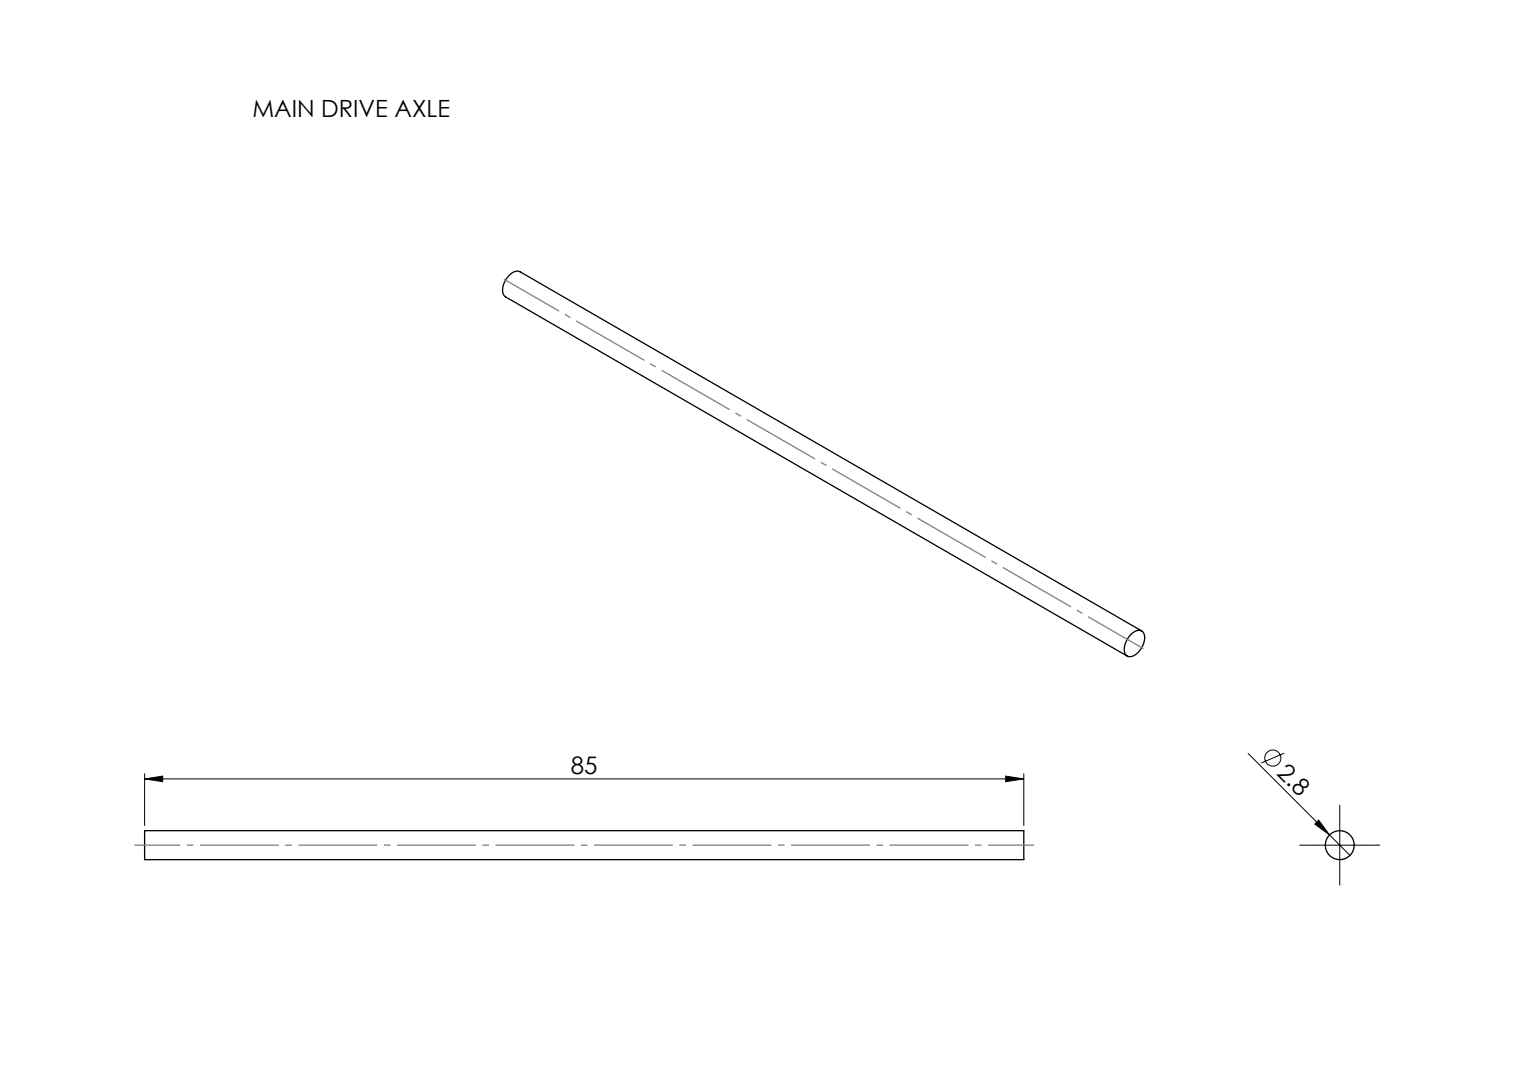
ISO-10303-21;
HEADER;
FILE_DESCRIPTION (('STEP AP214'),
    '1' );
FILE_NAME ('main drive axle.step',
    '2026-10-09T15:17:24',
    ( '' ),
    ( '' ),
    'SwSTEP 2.0',
    'SolidWorks 2026',
    '' );
FILE_SCHEMA (( 'AUTOMOTIVE_DESIGN' ));
ENDSEC;

DATA;
#499=ORIENTED_EDGE ( 'NONE', *, *, #57601, .F. ) ;
#808=LINE ( 'NONE', #11431, #63431 ) ;
#1848=CARTESIAN_POINT ( 'NONE',  ( 42.50000000000000000, -2.710505431213761085E-17, 1.201363017033314212E-18 ) ) ;
#2464=ORIENTED_EDGE ( 'NONE', *, *, #55323, .T. ) ;
#2684=( GEOMETRIC_REPRESENTATION_CONTEXT ( 3 ) GLOBAL_UNCERTAINTY_ASSIGNED_CONTEXT ( ( #8334 ) ) GLOBAL_UNIT_ASSIGNED_CONTEXT ( ( #22219, #27215, #7937 ) ) REPRESENTATION_CONTEXT ( 'NONE', 'WORKASPACE' ) );
#2711=CARTESIAN_POINT ( 'NONE',  ( -42.50000000000000000, 1.443454975684918283E-16, -1.399999999999999911 ) ) ;
#2771=CIRCLE ( 'NONE', #17659, 1.399999999999999911 ) ;
#5904=DIRECTION ( 'NONE',  ( 0.000000000000000000, 0.000000000000000000, 1.000000000000000000 ) ) ;
#7045=MANIFOLD_SOLID_BREP ( 'Boss-Extrude1', #36549 ) ;
#7247=SURFACE_SIDE_STYLE ('',( #33521 ) ) ;
#7363=AXIS2_PLACEMENT_3D ( 'NONE', #39531, #14261, #34541 ) ;
#7550=PRODUCT_DEFINITION ( 'UNKNOWN', '', #27136, #32561 ) ;
#7937=( NAMED_UNIT ( * ) SI_UNIT ( $, .STERADIAN. ) SOLID_ANGLE_UNIT ( ) );
#8334=UNCERTAINTY_MEASURE_WITH_UNIT (LENGTH_MEASURE( 1.000000000000000082E-05 ), #22219, 'distance_accuracy_value', 'NONE');
#8741=EDGE_LOOP ( 'NONE', ( #29240, #18346 ) ) ;
#10040=CARTESIAN_POINT ( 'NONE',  ( 0.000000000000000000, 0.000000000000000000, 0.000000000000000000 ) ) ;
#10513=CARTESIAN_POINT ( 'NONE',  ( 42.50000000000000000, -2.710505431213761085E-17, 1.201363017033314212E-18 ) ) ;
#10892=CARTESIAN_POINT ( 'NONE',  ( -42.50000000000000000, -2.710505431213761085E-17, 1.399999999999999911 ) ) ;
#11431=CARTESIAN_POINT ( 'NONE',  ( 42.50000000000000000, 1.443454975684918283E-16, -1.399999999999999911 ) ) ;
#11827=PRODUCT_CONTEXT ( 'NONE', #36599, 'mechanical' ) ;
#12138=DIRECTION ( 'NONE',  ( 0.000000000000000000, 0.000000000000000000, -1.000000000000000000 ) ) ;
#13237=FILL_AREA_STYLE ('',( #62779 ) ) ;
#13727=VERTEX_POINT ( 'NONE', #25182 ) ;
#14261=DIRECTION ( 'NONE',  ( 1.000000000000000000, 0.000000000000000000, 0.000000000000000000 ) ) ;
#14667=DIRECTION ( 'NONE',  ( 1.000000000000000000, 0.000000000000000000, 0.000000000000000000 ) ) ;
#15134=FILL_AREA_STYLE_COLOUR ( '', #41459 ) ;
#15352=DIRECTION ( 'NONE',  ( 0.000000000000000000, 0.000000000000000000, 1.000000000000000000 ) ) ;
#16037=AXIS2_PLACEMENT_3D ( 'NONE', #54307, #29028, #19381 ) ;
#16468=SURFACE_SIDE_STYLE ('',( #55724 ) ) ;
#16844=CIRCLE ( 'NONE', #31683, 1.399999999999999911 ) ;
#17031=STYLED_ITEM ( 'NONE', ( #38954 ), #7045 ) ;
#17072=APPLICATION_CONTEXT ( 'automotive_design' ) ;
#17513=MECHANICAL_DESIGN_GEOMETRIC_PRESENTATION_REPRESENTATION('',(#46184),#50457);
#17551=ORIENTED_EDGE ( 'NONE', *, *, #47305, .T. ) ;
#17659=AXIS2_PLACEMENT_3D ( 'NONE', #48672, #23390, #43659 ) ;
#18346=ORIENTED_EDGE ( 'NONE', *, *, #36575, .T. ) ;
#18597=ORIENTED_EDGE ( 'NONE', *, *, #36575, .F. ) ;
#18936=FACE_OUTER_BOUND ( 'NONE', #30270, .T. ) ;
#19015=PRODUCT ( 'main drive axle', 'main drive axle', '', ( #11827 ) ) ;
#19381=DIRECTION ( 'NONE',  ( 0.000000000000000000, 0.000000000000000000, 1.000000000000000000 ) ) ;
#19732=DIRECTION ( 'NONE',  ( 1.000000000000000000, 0.000000000000000000, 0.000000000000000000 ) ) ;
#21034=CIRCLE ( 'NONE', #58223, 1.399999999999999911 ) ;
#21449=( NAMED_UNIT ( * ) SI_UNIT ( $, .STERADIAN. ) SOLID_ANGLE_UNIT ( ) );
#22219=( LENGTH_UNIT ( ) NAMED_UNIT ( * ) SI_UNIT ( .MILLI., .METRE. ) );
#23012=DIRECTION ( 'NONE',  ( 0.000000000000000000, 0.000000000000000000, -1.000000000000000000 ) ) ;
#23129=SHAPE_DEFINITION_REPRESENTATION ( #64646, #25052 ) ;
#23192=VECTOR ( 'NONE', #27479, 1000.000000000000000 ) ;
#23390=DIRECTION ( 'NONE',  ( 1.000000000000000000, 0.000000000000000000, 0.000000000000000000 ) ) ;
#23405=( GEOMETRIC_REPRESENTATION_CONTEXT ( 3 ) GLOBAL_UNCERTAINTY_ASSIGNED_CONTEXT ( ( #62931 ) ) GLOBAL_UNIT_ASSIGNED_CONTEXT ( ( #53612, #46711, #21449 ) ) REPRESENTATION_CONTEXT ( 'NONE', 'WORKASPACE' ) );
#23639=UNCERTAINTY_MEASURE_WITH_UNIT (LENGTH_MEASURE( 1.000000000000000082E-05 ), #53809, 'distance_accuracy_value', 'NONE');
#24966=AXIS2_PLACEMENT_3D ( 'NONE', #10040, #15352, #14667 ) ;
#25052=SHAPE_REPRESENTATION ( 'main drive axle', ( #24966 ), #2684 ) ;
#25182=CARTESIAN_POINT ( 'NONE',  ( 42.50000000000000000, -2.710505431213761085E-17, 1.399999999999999911 ) ) ;
#25831=ORIENTED_EDGE ( 'NONE', *, *, #47305, .F. ) ;
#25837=FACE_OUTER_BOUND ( 'NONE', #39062, .T. ) ;
#26041=ORIENTED_EDGE ( 'NONE', *, *, #44633, .T. ) ;
#26449=DIRECTION ( 'NONE',  ( 1.000000000000000000, 0.000000000000000000, 0.000000000000000000 ) ) ;
#26837=CARTESIAN_POINT ( 'NONE',  ( 42.50000000000000000, -2.710505431213761085E-17, 1.399999999999999911 ) ) ;
#27136=PRODUCT_DEFINITION_FORMATION_WITH_SPECIFIED_SOURCE ( 'ANY', '', #19015, .NOT_KNOWN. ) ;
#27215=( NAMED_UNIT ( * ) PLANE_ANGLE_UNIT ( ) SI_UNIT ( $, .RADIAN. ) );
#27411=ADVANCED_FACE ( 'NONE', ( #59285 ), #33993, .T. ) ;
#27479=DIRECTION ( 'NONE',  ( -1.000000000000000000, -0.000000000000000000, -0.000000000000000000 ) ) ;
#27531=SURFACE_STYLE_USAGE ( .BOTH. , #7247 ) ;
#27537=AXIS2_PLACEMENT_3D ( 'NONE', #1848, #26449, #12138 ) ;
#27828=AXIS2_PLACEMENT_3D ( 'NONE', #58695, #33714, #37729 ) ;
#29028=DIRECTION ( 'NONE',  ( -1.000000000000000000, -0.000000000000000000, -0.000000000000000000 ) ) ;
#29240=ORIENTED_EDGE ( 'NONE', *, *, #30978, .T. ) ;
#29302=CARTESIAN_POINT ( 'NONE',  ( -42.50000000000000000, -2.710505431213761085E-17, 1.201363017033314212E-18 ) ) ;
#29902=ORIENTED_EDGE ( 'NONE', *, *, #30978, .F. ) ;
#29934=ORIENTED_EDGE ( 'NONE', *, *, #57601, .T. ) ;
#30270=EDGE_LOOP ( 'NONE', ( #59202, #499 ) ) ;
#30789=DIRECTION ( 'NONE',  ( -1.000000000000000000, -0.000000000000000000, -0.000000000000000000 ) ) ;
#30978=EDGE_CURVE ( 'NONE', #13727, #40874, #21034, .T. ) ;
#31683=AXIS2_PLACEMENT_3D ( 'NONE', #29302, #49595, #23012 ) ;
#32138=LINE ( 'NONE', #26837, #23192 ) ;
#32561=PRODUCT_DEFINITION_CONTEXT ( 'detailed design', #17072, 'design' ) ;
#33102=CARTESIAN_POINT ( 'NONE',  ( 42.50000000000000000, 1.443454975684918283E-16, -1.399999999999999911 ) ) ;
#33521=SURFACE_STYLE_FILL_AREA ( #13237 ) ;
#33695=ADVANCED_FACE ( 'NONE', ( #18936 ), #39200, .F. ) ;
#33714=DIRECTION ( 'NONE',  ( 1.000000000000000000, 0.000000000000000000, 0.000000000000000000 ) ) ;
#33894=ADVANCED_FACE ( 'NONE', ( #41745 ), #37075, .T. ) ;
#33993=CYLINDRICAL_SURFACE ( 'NONE', #16037, 1.399999999999999911 ) ;
#34541=DIRECTION ( 'NONE',  ( 0.000000000000000000, 0.000000000000000000, -1.000000000000000000 ) ) ;
#35208=VERTEX_POINT ( 'NONE', #10892 ) ;
#35320=DIRECTION ( 'NONE',  ( 0.000000000000000000, 0.000000000000000000, -1.000000000000000000 ) ) ;
#35417=FILL_AREA_STYLE ('',( #15134 ) ) ;
#36549=CLOSED_SHELL ( 'NONE', ( #44276, #27411, #33894, #33695 ) ) ;
#36575=EDGE_CURVE ( 'NONE', #40874, #13727, #42661, .T. ) ;
#36599=APPLICATION_CONTEXT ( 'automotive_design' ) ;
#37075=PLANE ( 'NONE',  #27537 ) ;
#37239=ADVANCED_BREP_SHAPE_REPRESENTATION ( '', ( #7045, #24966 ), #2684 ) ;
#37729=DIRECTION ( 'NONE',  ( 0.000000000000000000, 0.000000000000000000, -1.000000000000000000 ) ) ;
#38954=PRESENTATION_STYLE_ASSIGNMENT (( #63545 ) ) ;
#39062=EDGE_LOOP ( 'NONE', ( #18597, #26041, #29934, #25831 ) ) ;
#39200=PLANE ( 'NONE',  #7363 ) ;
#39425=ORIENTED_EDGE ( 'NONE', *, *, #44633, .F. ) ;
#39531=CARTESIAN_POINT ( 'NONE',  ( -42.50000000000000000, -2.710505431213761085E-17, 1.201363017033314212E-18 ) ) ;
#40874=VERTEX_POINT ( 'NONE', #33102 ) ;
#41355=DIRECTION ( 'NONE',  ( -1.000000000000000000, -0.000000000000000000, -0.000000000000000000 ) ) ;
#41459=COLOUR_RGB ( '', 0.66274510, 0.83137255, 0.94901961) ;
#41745=FACE_OUTER_BOUND ( 'NONE', #8741, .T. ) ;
#41935=COLOUR_RGB ( '', 0.66274510, 0.83137255, 0.94901961) ;
#42157=( NAMED_UNIT ( * ) PLANE_ANGLE_UNIT ( ) SI_UNIT ( $, .RADIAN. ) );
#42661=CIRCLE ( 'NONE', #27828, 1.399999999999999911 ) ;
#43150=SHAPE_REPRESENTATION_RELATIONSHIP ( 'NONE' , 'NONE' ,  #25052, #37239 ) ;
#43659=DIRECTION ( 'NONE',  ( 0.000000000000000000, 0.000000000000000000, -1.000000000000000000 ) ) ;
#44276=ADVANCED_FACE ( 'NONE', ( #25837 ), #56076, .T. ) ;
#44633=EDGE_CURVE ( 'NONE', #40874, #51496, #808, .T. ) ;
#46184=STYLED_ITEM ( 'NONE', ( #47508 ), #37239 ) ;
#46711=( NAMED_UNIT ( * ) PLANE_ANGLE_UNIT ( ) SI_UNIT ( $, .RADIAN. ) );
#47305=EDGE_CURVE ( 'NONE', #13727, #35208, #32138, .T. ) ;
#47508=PRESENTATION_STYLE_ASSIGNMENT (( #27531 ) ) ;
#48196=EDGE_LOOP ( 'NONE', ( #39425, #29902, #17551, #2464 ) ) ;
#48611=AXIS2_PLACEMENT_3D ( 'NONE', #10513, #30789, #5904 ) ;
#48672=CARTESIAN_POINT ( 'NONE',  ( -42.50000000000000000, -2.710505431213761085E-17, 1.201363017033314212E-18 ) ) ;
#49595=DIRECTION ( 'NONE',  ( 1.000000000000000000, 0.000000000000000000, 0.000000000000000000 ) ) ;
#50457=( GEOMETRIC_REPRESENTATION_CONTEXT ( 3 ) GLOBAL_UNCERTAINTY_ASSIGNED_CONTEXT ( ( #23639 ) ) GLOBAL_UNIT_ASSIGNED_CONTEXT ( ( #53809, #42157, #62445 ) ) REPRESENTATION_CONTEXT ( 'NONE', 'WORKASPACE' ) );
#51496=VERTEX_POINT ( 'NONE', #2711 ) ;
#53612=( LENGTH_UNIT ( ) NAMED_UNIT ( * ) SI_UNIT ( .MILLI., .METRE. ) );
#53809=( LENGTH_UNIT ( ) NAMED_UNIT ( * ) SI_UNIT ( .MILLI., .METRE. ) );
#54307=CARTESIAN_POINT ( 'NONE',  ( 42.50000000000000000, -2.710505431213761085E-17, 1.201363017033314212E-18 ) ) ;
#55323=EDGE_CURVE ( 'NONE', #35208, #51496, #2771, .T. ) ;
#55724=SURFACE_STYLE_FILL_AREA ( #35417 ) ;
#56076=CYLINDRICAL_SURFACE ( 'NONE', #48611, 1.399999999999999911 ) ;
#57383=MECHANICAL_DESIGN_GEOMETRIC_PRESENTATION_REPRESENTATION('',(#17031),#23405);
#57601=EDGE_CURVE ( 'NONE', #51496, #35208, #16844, .T. ) ;
#58223=AXIS2_PLACEMENT_3D ( 'NONE', #65267, #19732, #35320 ) ;
#58695=CARTESIAN_POINT ( 'NONE',  ( 42.50000000000000000, -2.710505431213761085E-17, 1.201363017033314212E-18 ) ) ;
#59202=ORIENTED_EDGE ( 'NONE', *, *, #55323, .F. ) ;
#59285=FACE_OUTER_BOUND ( 'NONE', #48196, .T. ) ;
#62445=( NAMED_UNIT ( * ) SI_UNIT ( $, .STERADIAN. ) SOLID_ANGLE_UNIT ( ) );
#62779=FILL_AREA_STYLE_COLOUR ( '', #41935 ) ;
#62931=UNCERTAINTY_MEASURE_WITH_UNIT (LENGTH_MEASURE( 1.000000000000000082E-05 ), #53612, 'distance_accuracy_value', 'NONE');
#63431=VECTOR ( 'NONE', #41355, 1000.000000000000000 ) ;
#63545=SURFACE_STYLE_USAGE ( .BOTH. , #16468 ) ;
#64646=PRODUCT_DEFINITION_SHAPE ( 'NONE', 'NONE',  #7550 ) ;
#65267=CARTESIAN_POINT ( 'NONE',  ( 42.50000000000000000, -2.710505431213761085E-17, 1.201363017033314212E-18 ) ) ;
ENDSEC;
END-ISO-10303-21;
